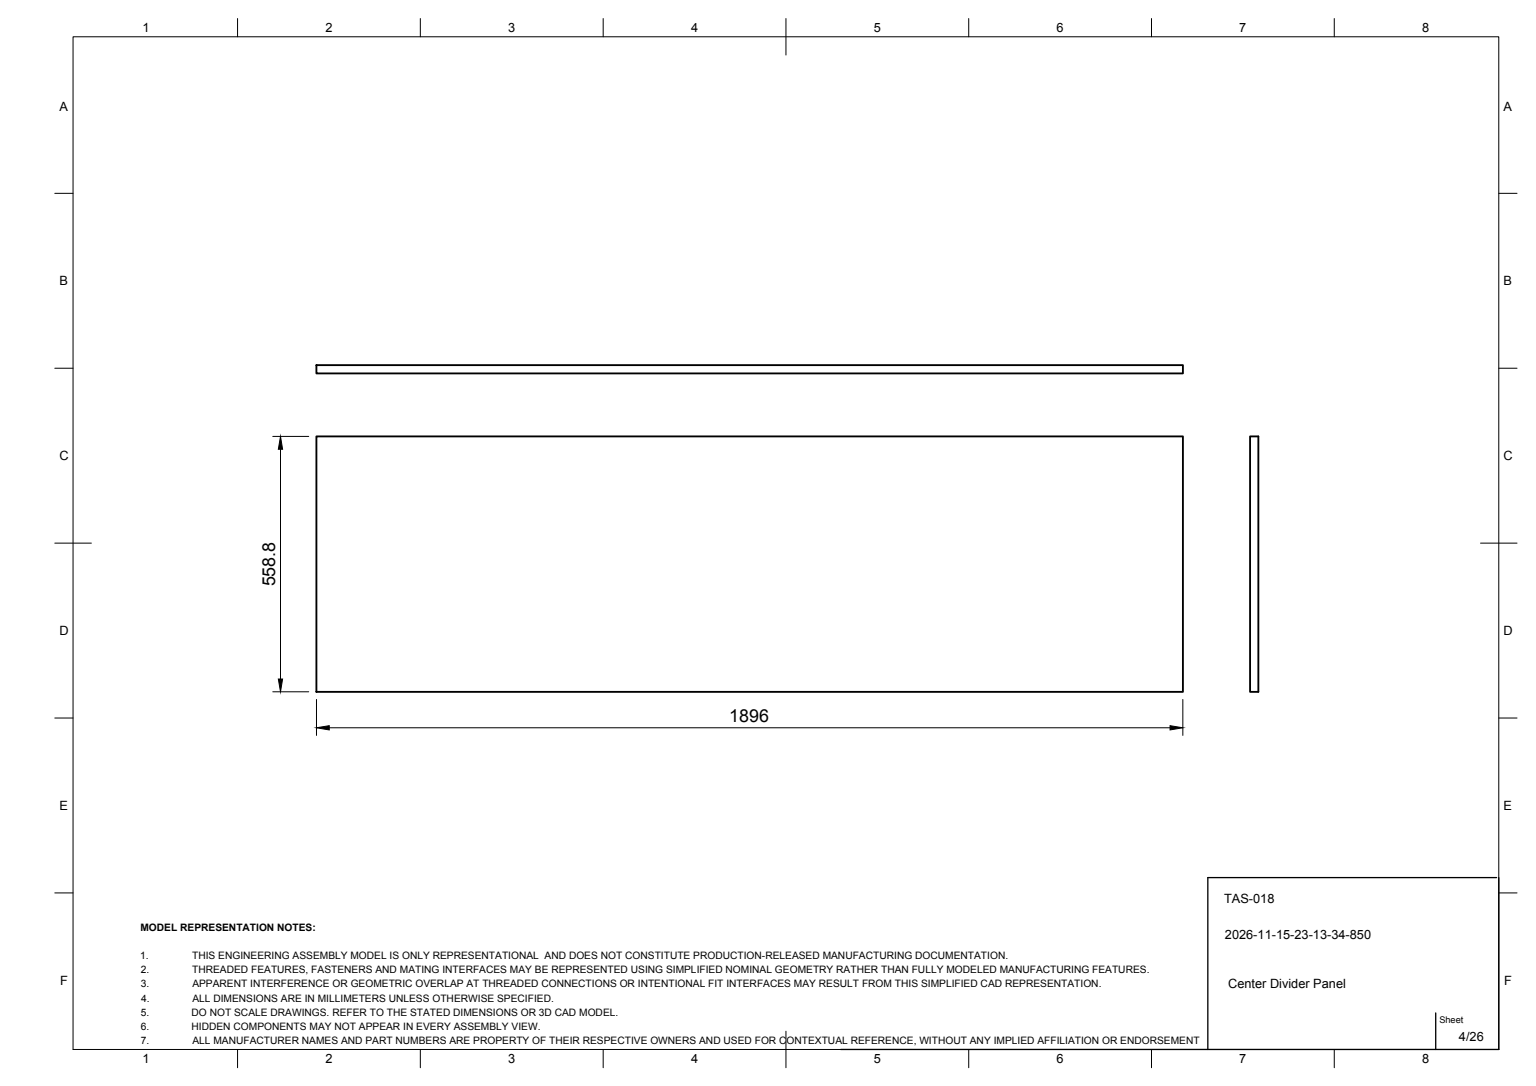
ISO-10303-21;
HEADER;
/* Generated by software containing ST-Developer
 * from STEP Tools, Inc. (www.steptools.com) 
 */

FILE_DESCRIPTION(
/* description */ (''),
/* implementation_level */ '2;1');

FILE_NAME(
/* name */ 'Center Divider Panel.step',
/* time_stamp */ '2026-11-15T15:17:57-08:00',
/* author */ (''),
/* organization */ (''),
/* preprocessor_version */ 'ST-DEVELOPER v20.2',
/* originating_system */ 'Autodesk Translation Framework v15.17.0.0',
/* authorisation */ '');

FILE_SCHEMA (('AUTOMOTIVE_DESIGN { 1 0 10303 214 3 1 1 }'));
ENDSEC;

DATA;
#10=MECHANICAL_DESIGN_GEOMETRIC_PRESENTATION_REPRESENTATION('',(#179),#3723);
#131=SHAPE_REPRESENTATION_RELATIONSHIP('SRR','None',#3812,#155);
#155=ADVANCED_BREP_SHAPE_REPRESENTATION('',(#203),#3701);
#179=STYLED_ITEM('',(#3943),#203);
#203=MANIFOLD_SOLID_BREP('Body1',#2027);
#237=FACE_OUTER_BOUND('',#363,.T.);
#238=FACE_OUTER_BOUND('',#364,.T.);
#239=FACE_OUTER_BOUND('',#365,.T.);
#240=FACE_OUTER_BOUND('',#366,.T.);
#241=FACE_OUTER_BOUND('',#367,.T.);
#242=FACE_OUTER_BOUND('',#368,.T.);
#363=EDGE_LOOP('',(#1359,#1360,#1361,#1362));
#364=EDGE_LOOP('',(#1363,#1364,#1365,#1366));
#365=EDGE_LOOP('',(#1367,#1368,#1369,#1370));
#366=EDGE_LOOP('',(#1371,#1372,#1373,#1374));
#367=EDGE_LOOP('',(#1375,#1376,#1377,#1378));
#368=EDGE_LOOP('',(#1379,#1380,#1381,#1382));
#501=LINE('',#3164,#723);
#502=LINE('',#3166,#724);
#503=LINE('',#3168,#725);
#504=LINE('',#3169,#726);
#505=LINE('',#3172,#727);
#506=LINE('',#3174,#728);
#507=LINE('',#3175,#729);
#508=LINE('',#3178,#730);
#509=LINE('',#3180,#731);
#510=LINE('',#3181,#732);
#511=LINE('',#3183,#733);
#512=LINE('',#3184,#734);
#723=VECTOR('',#2565,74.6456692913386);
#724=VECTOR('',#2566,22.);
#725=VECTOR('',#2567,74.6456692913386);
#726=VECTOR('',#2568,22.);
#727=VECTOR('',#2571,0.708661417322835);
#728=VECTOR('',#2572,22.);
#729=VECTOR('',#2573,0.708661417322835);
#730=VECTOR('',#2576,74.6456692913386);
#731=VECTOR('',#2577,22.);
#732=VECTOR('',#2578,74.6456692913386);
#733=VECTOR('',#2581,0.708661417322835);
#734=VECTOR('',#2582,0.708661417322835);
#937=VERTEX_POINT('',#3162);
#938=VERTEX_POINT('',#3163);
#939=VERTEX_POINT('',#3165);
#940=VERTEX_POINT('',#3167);
#941=VERTEX_POINT('',#3171);
#942=VERTEX_POINT('',#3173);
#943=VERTEX_POINT('',#3177);
#944=VERTEX_POINT('',#3179);
#1101=EDGE_CURVE('',#937,#938,#501,.T.);
#1102=EDGE_CURVE('',#939,#938,#502,.T.);
#1103=EDGE_CURVE('',#940,#939,#503,.T.);
#1104=EDGE_CURVE('',#940,#937,#504,.T.);
#1105=EDGE_CURVE('',#938,#941,#505,.T.);
#1106=EDGE_CURVE('',#942,#941,#506,.T.);
#1107=EDGE_CURVE('',#939,#942,#507,.T.);
#1108=EDGE_CURVE('',#941,#943,#508,.T.);
#1109=EDGE_CURVE('',#944,#943,#509,.T.);
#1110=EDGE_CURVE('',#942,#944,#510,.T.);
#1111=EDGE_CURVE('',#943,#937,#511,.T.);
#1112=EDGE_CURVE('',#944,#940,#512,.T.);
#1359=ORIENTED_EDGE('',*,*,#1101,.T.);
#1360=ORIENTED_EDGE('',*,*,#1102,.F.);
#1361=ORIENTED_EDGE('',*,*,#1103,.F.);
#1362=ORIENTED_EDGE('',*,*,#1104,.T.);
#1363=ORIENTED_EDGE('',*,*,#1105,.T.);
#1364=ORIENTED_EDGE('',*,*,#1106,.F.);
#1365=ORIENTED_EDGE('',*,*,#1107,.F.);
#1366=ORIENTED_EDGE('',*,*,#1102,.T.);
#1367=ORIENTED_EDGE('',*,*,#1108,.T.);
#1368=ORIENTED_EDGE('',*,*,#1109,.F.);
#1369=ORIENTED_EDGE('',*,*,#1110,.F.);
#1370=ORIENTED_EDGE('',*,*,#1106,.T.);
#1371=ORIENTED_EDGE('',*,*,#1111,.T.);
#1372=ORIENTED_EDGE('',*,*,#1104,.F.);
#1373=ORIENTED_EDGE('',*,*,#1112,.F.);
#1374=ORIENTED_EDGE('',*,*,#1109,.T.);
#1375=ORIENTED_EDGE('',*,*,#1103,.T.);
#1376=ORIENTED_EDGE('',*,*,#1107,.T.);
#1377=ORIENTED_EDGE('',*,*,#1110,.T.);
#1378=ORIENTED_EDGE('',*,*,#1112,.T.);
#1379=ORIENTED_EDGE('',*,*,#1101,.F.);
#1380=ORIENTED_EDGE('',*,*,#1111,.F.);
#1381=ORIENTED_EDGE('',*,*,#1108,.F.);
#1382=ORIENTED_EDGE('',*,*,#1105,.F.);
#1791=PLANE('',#2332);
#1792=PLANE('',#2333);
#1793=PLANE('',#2334);
#1794=PLANE('',#2335);
#1795=PLANE('',#2336);
#1796=PLANE('',#2337);
#1911=ADVANCED_FACE('',(#237),#1791,.F.);
#1912=ADVANCED_FACE('',(#238),#1792,.F.);
#1913=ADVANCED_FACE('',(#239),#1793,.F.);
#1914=ADVANCED_FACE('',(#240),#1794,.F.);
#1915=ADVANCED_FACE('',(#241),#1795,.T.);
#1916=ADVANCED_FACE('',(#242),#1796,.F.);
#2027=CLOSED_SHELL('',(#1911,#1912,#1913,#1914,#1915,#1916));
#2331=AXIS2_PLACEMENT_3D('',#3160,#2561,#2562);
#2332=AXIS2_PLACEMENT_3D('',#3161,#2563,#2564);
#2333=AXIS2_PLACEMENT_3D('',#3170,#2569,#2570);
#2334=AXIS2_PLACEMENT_3D('',#3176,#2574,#2575);
#2335=AXIS2_PLACEMENT_3D('',#3182,#2579,#2580);
#2336=AXIS2_PLACEMENT_3D('',#3185,#2583,#2584);
#2337=AXIS2_PLACEMENT_3D('',#3186,#2585,#2586);
#2561=DIRECTION('axis',(0.,0.,1.));
#2562=DIRECTION('refdir',(1.,0.,0.));
#2563=DIRECTION('center_axis',(1.,3.05589473088741E-16,0.));
#2564=DIRECTION('ref_axis',(0.,0.,-1.));
#2565=DIRECTION('',(3.05662668172116E-16,-1.,0.));
#2566=DIRECTION('',(0.,0.,-1.));
#2567=DIRECTION('',(3.05662668172116E-16,-1.,0.));
#2568=DIRECTION('',(0.,0.,-1.));
#2569=DIRECTION('center_axis',(0.,1.,0.));
#2570=DIRECTION('ref_axis',(0.,0.,1.));
#2571=DIRECTION('',(1.,0.,0.));
#2572=DIRECTION('',(0.,0.,-1.));
#2573=DIRECTION('',(1.,0.,0.));
#2574=DIRECTION('center_axis',(-1.,-3.05589473088741E-16,0.));
#2575=DIRECTION('ref_axis',(0.,0.,1.));
#2576=DIRECTION('',(-3.05662668172116E-16,1.,0.));
#2577=DIRECTION('',(0.,0.,-1.));
#2578=DIRECTION('',(-3.05662668172116E-16,1.,0.));
#2579=DIRECTION('center_axis',(0.,-1.,0.));
#2580=DIRECTION('ref_axis',(0.,0.,-1.));
#2581=DIRECTION('',(-1.,0.,0.));
#2582=DIRECTION('',(-1.,0.,0.));
#2583=DIRECTION('center_axis',(0.,0.,1.));
#2584=DIRECTION('ref_axis',(1.,0.,0.));
#2585=DIRECTION('center_axis',(0.,0.,1.));
#2586=DIRECTION('ref_axis',(1.,0.,0.));
#3160=CARTESIAN_POINT('',(0.,0.,0.));
#3161=CARTESIAN_POINT('Origin',(-0.354330708661419,4.64566929133858,22.));
#3162=CARTESIAN_POINT('',(-0.354330708661442,79.2913385826772,0.));
#3163=CARTESIAN_POINT('',(-0.354330708661419,4.64566929133858,0.));
#3164=CARTESIAN_POINT('',(-0.354330708661442,79.2913385826772,0.));
#3165=CARTESIAN_POINT('',(-0.354330708661419,4.64566929133858,22.));
#3166=CARTESIAN_POINT('',(-0.354330708661419,4.64566929133858,22.));
#3167=CARTESIAN_POINT('',(-0.354330708661442,79.2913385826772,22.));
#3168=CARTESIAN_POINT('',(-0.354330708661442,79.2913385826772,22.));
#3169=CARTESIAN_POINT('',(-0.354330708661442,79.2913385826772,22.));
#3170=CARTESIAN_POINT('Origin',(0.354330708661416,4.64566929133858,22.));
#3171=CARTESIAN_POINT('',(0.354330708661416,4.64566929133858,0.));
#3172=CARTESIAN_POINT('',(-0.354330708661419,4.64566929133858,0.));
#3173=CARTESIAN_POINT('',(0.354330708661416,4.64566929133858,22.));
#3174=CARTESIAN_POINT('',(0.354330708661416,4.64566929133858,22.));
#3175=CARTESIAN_POINT('',(-0.354330708661419,4.64566929133858,22.));
#3176=CARTESIAN_POINT('Origin',(0.354330708661416,4.64566929133858,22.));
#3177=CARTESIAN_POINT('',(0.354330708661393,79.2913385826772,0.));
#3178=CARTESIAN_POINT('',(0.354330708661416,4.64566929133858,0.));
#3179=CARTESIAN_POINT('',(0.354330708661393,79.2913385826772,22.));
#3180=CARTESIAN_POINT('',(0.354330708661393,79.2913385826772,22.));
#3181=CARTESIAN_POINT('',(0.354330708661416,4.64566929133858,22.));
#3182=CARTESIAN_POINT('Origin',(0.354330708661393,79.2913385826772,22.));
#3183=CARTESIAN_POINT('',(0.354330708661393,79.2913385826772,0.));
#3184=CARTESIAN_POINT('',(0.354330708661393,79.2913385826772,22.));
#3185=CARTESIAN_POINT('Origin',(0.,0.,22.));
#3186=CARTESIAN_POINT('Origin',(0.,0.,0.));
#3674=UNCERTAINTY_MEASURE_WITH_UNIT(LENGTH_MEASURE(0.000393700787401575),
#3725,'DISTANCE_ACCURACY_VALUE',
'Maximum model space distance between geometric entities at asserted c
onnectivities');
#3696=UNCERTAINTY_MEASURE_WITH_UNIT(LENGTH_MEASURE(0.000393700787401575),
#3725,'DISTANCE_ACCURACY_VALUE',
'Maximum model space distance between geometric entities at asserted c
onnectivities');
#3701=(
GEOMETRIC_REPRESENTATION_CONTEXT(3)
GLOBAL_UNCERTAINTY_ASSIGNED_CONTEXT((#3674))
GLOBAL_UNIT_ASSIGNED_CONTEXT((#3725,#3729,#3730))
REPRESENTATION_CONTEXT('','3D')
);
#3723=(
GEOMETRIC_REPRESENTATION_CONTEXT(3)
GLOBAL_UNCERTAINTY_ASSIGNED_CONTEXT((#3696))
GLOBAL_UNIT_ASSIGNED_CONTEXT((#3725,#3729,#3730))
REPRESENTATION_CONTEXT('','3D')
);
#3724=DIMENSIONAL_EXPONENTS(1.,0.,0.,0.,0.,0.,0.);
#3725=(
CONVERSION_BASED_UNIT('inch',#3728)
LENGTH_UNIT()
NAMED_UNIT(#3724)
);
#3726=(
LENGTH_UNIT()
NAMED_UNIT(*)
SI_UNIT(.MILLI.,.METRE.)
);
#3728=LENGTH_MEASURE_WITH_UNIT(LENGTH_MEASURE(25.4),#3726);
#3729=(
NAMED_UNIT(*)
PLANE_ANGLE_UNIT()
SI_UNIT($,.RADIAN.)
);
#3730=(
NAMED_UNIT(*)
SI_UNIT($,.STERADIAN.)
SOLID_ANGLE_UNIT()
);
#3735=SHAPE_DEFINITION_REPRESENTATION(#3762,#3812);
#3762=PRODUCT_DEFINITION_SHAPE('',$,#3839);
#3812=SHAPE_REPRESENTATION('',(#2331),#3701);
#3834=PRODUCT_DEFINITION_CONTEXT('part definition',#3914,'design');
#3839=PRODUCT_DEFINITION('2026-11-15-23-13-34-850',
'Center Divider Panel',#3865,#3834);
#3865=PRODUCT_DEFINITION_FORMATION('',$,#3920);
#3914=APPLICATION_CONTEXT(
'Core Data for Automotive Mechanical Design Process');
#3915=PRODUCT_CONTEXT('part definition',#3914,'mechanical');
#3920=PRODUCT('2026-11-15-23-13-34-850','Center Divider Panel',$,(#3915));
#3943=PRESENTATION_STYLE_ASSIGNMENT((#3951));
#3951=SURFACE_STYLE_USAGE(.BOTH.,#3959);
#3959=SURFACE_SIDE_STYLE('',(#3967));
#3967=SURFACE_STYLE_FILL_AREA(#3975);
#3975=FILL_AREA_STYLE('Dark Blue',(#3983));
#3983=FILL_AREA_STYLE_COLOUR('Dark Blue',#3991);
#3991=COLOUR_RGB('Dark Blue',0.,0.125490196078431,0.376470588235294);
ENDSEC;
END-ISO-10303-21;
